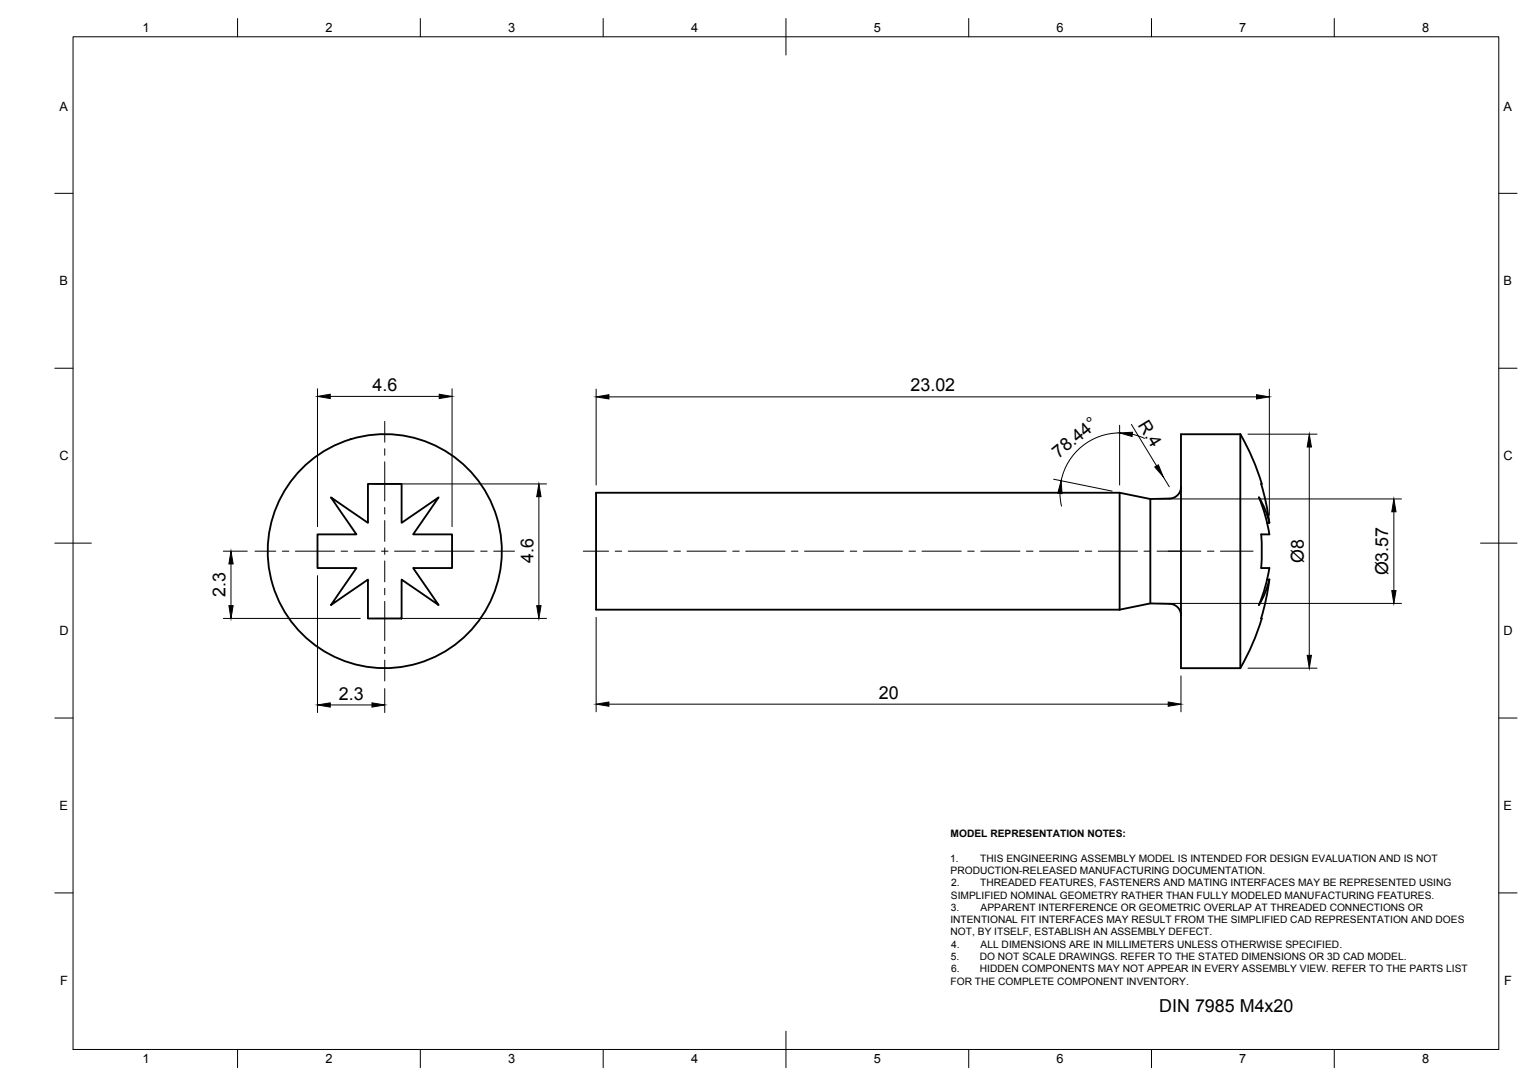
ISO-10303-21;
HEADER;
/* Generated by software containing ST-Developer
 * from STEP Tools, Inc. (www.steptools.com) 
 */

FILE_DESCRIPTION(
/* description */ ('STEP AP214'),
/* implementation_level */ '2;1');

FILE_NAME(
/* name */ 'DIN 7985 M4x20.step',
/* time_stamp */ '2026-10-07T12:18:07-07:00',
/* author */ (''),
/* organization */ (''),
/* preprocessor_version */ 'ST-DEVELOPER v20.2',
/* originating_system */ 'Autodesk Translation Framework v15.15.0.0',
/* authorisation */ '');

FILE_SCHEMA (('AUTOMOTIVE_DESIGN { 1 0 10303 214 3 1 1 }'));
ENDSEC;

DATA;
#10=MECHANICAL_DESIGN_GEOMETRIC_PRESENTATION_REPRESENTATION('',(#123),#62974);
#79=SPHERICAL_SURFACE('',#15475,8.00000000000091);
#99=SHAPE_REPRESENTATION_RELATIONSHIP('SRR','None',#63022,#111);
#111=ADVANCED_BREP_SHAPE_REPRESENTATION('',(#135),#62963);
#123=STYLED_ITEM('',(#63090),#135);
#135=MANIFOLD_SOLID_BREP('Body1',#15193);
#210=FACE_BOUND('',#4662,.T.);
#211=FACE_BOUND('',#4669,.T.);
#342=PLANE('',#15508);
#343=PLANE('',#15509);
#344=PLANE('',#15510);
#345=PLANE('',#15511);
#346=PLANE('',#15512);
#347=PLANE('',#15513);
#348=PLANE('',#15514);
#349=PLANE('',#15515);
#350=PLANE('',#15516);
#351=PLANE('',#15517);
#352=PLANE('',#15518);
#353=PLANE('',#15519);
#354=PLANE('',#15520);
#355=PLANE('',#15521);
#356=PLANE('',#15522);
#357=PLANE('',#15523);
#358=PLANE('',#15524);
#359=PLANE('',#15525);
#360=PLANE('',#15526);
#361=PLANE('',#15527);
#362=PLANE('',#15528);
#363=PLANE('',#15529);
#364=PLANE('',#15530);
#1035=CONICAL_SURFACE('',#15500,1.8001015361136,0.0225322446275356);
#1036=CONICAL_SURFACE('',#15503,1.78525,0.201741568445237);
#1193=LINE('',#33921,#2386);
#1194=LINE('',#33972,#2387);
#1195=LINE('',#33980,#2388);
#1196=LINE('',#33985,#2389);
#1197=LINE('',#33990,#2390);
#1198=LINE('',#33992,#2391);
#1199=LINE('',#33993,#2392);
#1200=LINE('',#33997,#2393);
#1201=LINE('',#33998,#2394);
#1202=LINE('',#33999,#2395);
#1203=LINE('',#34002,#2396);
#1204=LINE('',#34003,#2397);
#1205=LINE('',#34006,#2398);
#1206=LINE('',#34007,#2399);
#1207=LINE('',#34010,#2400);
#1208=LINE('',#34011,#2401);
#1209=LINE('',#34014,#2402);
#1210=LINE('',#34015,#2403);
#1211=LINE('',#34018,#2404);
#1212=LINE('',#34019,#2405);
#1213=LINE('',#34022,#2406);
#1214=LINE('',#34023,#2407);
#1215=LINE('',#34026,#2408);
#1216=LINE('',#34027,#2409);
#1217=LINE('',#34030,#2410);
#1218=LINE('',#34031,#2411);
#1219=LINE('',#34034,#2412);
#1220=LINE('',#34035,#2413);
#1221=LINE('',#34038,#2414);
#1222=LINE('',#34039,#2415);
#1223=LINE('',#34042,#2416);
#1224=LINE('',#34043,#2417);
#1225=LINE('',#34046,#2418);
#1226=LINE('',#34047,#2419);
#1227=LINE('',#34050,#2420);
#1228=LINE('',#34051,#2421);
#1229=LINE('',#34054,#2422);
#1230=LINE('',#34055,#2423);
#1231=LINE('',#34058,#2424);
#1232=LINE('',#34059,#2425);
#1233=LINE('',#34061,#2426);
#1234=LINE('',#34064,#2427);
#1235=LINE('',#34065,#2428);
#1236=LINE('',#34067,#2429);
#2386=VECTOR('',#17366,4.);
#2387=VECTOR('',#17421,1.8001015361136);
#2388=VECTOR('',#17430,1.78525);
#2389=VECTOR('',#17437,2.);
#2390=VECTOR('',#17444,1000.);
#2391=VECTOR('',#17445,1000.);
#2392=VECTOR('',#17446,1000.);
#2393=VECTOR('',#17449,1000.);
#2394=VECTOR('',#17450,1000.);
#2395=VECTOR('',#17451,1000.);
#2396=VECTOR('',#17454,1000.);
#2397=VECTOR('',#17455,1000.);
#2398=VECTOR('',#17458,1000.);
#2399=VECTOR('',#17459,1000.);
#2400=VECTOR('',#17462,1000.);
#2401=VECTOR('',#17463,1000.);
#2402=VECTOR('',#17466,1000.);
#2403=VECTOR('',#17467,1000.);
#2404=VECTOR('',#17470,1000.);
#2405=VECTOR('',#17471,1000.);
#2406=VECTOR('',#17474,1000.);
#2407=VECTOR('',#17475,1000.);
#2408=VECTOR('',#17478,1000.);
#2409=VECTOR('',#17479,1000.);
#2410=VECTOR('',#17482,1000.);
#2411=VECTOR('',#17483,1000.);
#2412=VECTOR('',#17486,1000.);
#2413=VECTOR('',#17487,1000.);
#2414=VECTOR('',#17490,1000.);
#2415=VECTOR('',#17491,1000.);
#2416=VECTOR('',#17494,1000.);
#2417=VECTOR('',#17495,1000.);
#2418=VECTOR('',#17498,1000.);
#2419=VECTOR('',#17499,1000.);
#2420=VECTOR('',#17502,1000.);
#2421=VECTOR('',#17503,1000.);
#2422=VECTOR('',#17506,1000.);
#2423=VECTOR('',#17507,1000.);
#2424=VECTOR('',#17510,1000.);
#2425=VECTOR('',#17511,1000.);
#2426=VECTOR('',#17514,1000.);
#2427=VECTOR('',#17517,1000.);
#2428=VECTOR('',#17518,1000.);
#2429=VECTOR('',#17521,1000.);
#3459=CYLINDRICAL_SURFACE('',#15472,4.);
#3460=CYLINDRICAL_SURFACE('',#15506,2.);
#3777=FACE_OUTER_BOUND('',#4660,.T.);
#3778=FACE_OUTER_BOUND('',#4661,.T.);
#3779=FACE_OUTER_BOUND('',#4663,.T.);
#3780=FACE_OUTER_BOUND('',#4664,.T.);
#3781=FACE_OUTER_BOUND('',#4665,.T.);
#3782=FACE_OUTER_BOUND('',#4666,.T.);
#3783=FACE_OUTER_BOUND('',#4667,.T.);
#3784=FACE_OUTER_BOUND('',#4668,.T.);
#3785=FACE_OUTER_BOUND('',#4670,.T.);
#3786=FACE_OUTER_BOUND('',#4671,.T.);
#3787=FACE_OUTER_BOUND('',#4672,.T.);
#3788=FACE_OUTER_BOUND('',#4673,.T.);
#3789=FACE_OUTER_BOUND('',#4674,.T.);
#3790=FACE_OUTER_BOUND('',#4675,.T.);
#3791=FACE_OUTER_BOUND('',#4676,.T.);
#3792=FACE_OUTER_BOUND('',#4677,.T.);
#3793=FACE_OUTER_BOUND('',#4678,.T.);
#3794=FACE_OUTER_BOUND('',#4679,.T.);
#3795=FACE_OUTER_BOUND('',#4680,.T.);
#3796=FACE_OUTER_BOUND('',#4681,.T.);
#3797=FACE_OUTER_BOUND('',#4682,.T.);
#3798=FACE_OUTER_BOUND('',#4683,.T.);
#3799=FACE_OUTER_BOUND('',#4684,.T.);
#3800=FACE_OUTER_BOUND('',#4685,.T.);
#3801=FACE_OUTER_BOUND('',#4686,.T.);
#3802=FACE_OUTER_BOUND('',#4687,.T.);
#3803=FACE_OUTER_BOUND('',#4688,.T.);
#3804=FACE_OUTER_BOUND('',#4689,.T.);
#3805=FACE_OUTER_BOUND('',#4690,.T.);
#4660=EDGE_LOOP('',(#10207,#10208,#10209,#10210));
#4661=EDGE_LOOP('',(#10211));
#4662=EDGE_LOOP('',(#10212,#10213,#10214,#10215,#10216,#10217,#10218,#10219,
#10220,#10221,#10222,#10223,#10224,#10225,#10226,#10227,#10228,#10229,#10230,
#10231));
#4663=EDGE_LOOP('',(#10232,#10233,#10234,#10235));
#4664=EDGE_LOOP('',(#10236,#10237,#10238,#10239,#10240));
#4665=EDGE_LOOP('',(#10241,#10242,#10243,#10244,#10245,#10246));
#4666=EDGE_LOOP('',(#10247,#10248,#10249,#10250,#10251));
#4667=EDGE_LOOP('',(#10252));
#4668=EDGE_LOOP('',(#10253));
#4669=EDGE_LOOP('',(#10254));
#4670=EDGE_LOOP('',(#10255,#10256,#10257,#10258));
#4671=EDGE_LOOP('',(#10259,#10260,#10261,#10262));
#4672=EDGE_LOOP('',(#10263,#10264,#10265,#10266));
#4673=EDGE_LOOP('',(#10267,#10268,#10269,#10270));
#4674=EDGE_LOOP('',(#10271,#10272,#10273,#10274));
#4675=EDGE_LOOP('',(#10275,#10276,#10277,#10278));
#4676=EDGE_LOOP('',(#10279,#10280,#10281,#10282));
#4677=EDGE_LOOP('',(#10283,#10284,#10285,#10286));
#4678=EDGE_LOOP('',(#10287,#10288,#10289,#10290));
#4679=EDGE_LOOP('',(#10291,#10292,#10293,#10294));
#4680=EDGE_LOOP('',(#10295,#10296,#10297,#10298));
#4681=EDGE_LOOP('',(#10299,#10300,#10301,#10302));
#4682=EDGE_LOOP('',(#10303,#10304,#10305,#10306));
#4683=EDGE_LOOP('',(#10307,#10308,#10309,#10310));
#4684=EDGE_LOOP('',(#10311,#10312,#10313,#10314));
#4685=EDGE_LOOP('',(#10315,#10316,#10317,#10318));
#4686=EDGE_LOOP('',(#10319,#10320,#10321,#10322));
#4687=EDGE_LOOP('',(#10323,#10324,#10325,#10326));
#4688=EDGE_LOOP('',(#10327,#10328,#10329,#10330,#10331,#10332,#10333,#10334,
#10335,#10336,#10337,#10338,#10339,#10340,#10341,#10342,#10343,#10344,#10345,
#10346));
#4689=EDGE_LOOP('',(#10347,#10348,#10349,#10350));
#4690=EDGE_LOOP('',(#10351,#10352,#10353,#10354));
#5553=CIRCLE('',#15473,4.);
#5554=CIRCLE('',#15474,4.);
#5555=CIRCLE('',#15476,7.66224510179708);
#5556=CIRCLE('',#15477,7.97930918062551);
#5557=CIRCLE('',#15478,7.98595584236444);
#5558=CIRCLE('',#15479,7.98595584236446);
#5559=CIRCLE('',#15480,7.97930918062549);
#5560=CIRCLE('',#15481,7.66224510179716);
#5561=CIRCLE('',#15482,7.97930918062553);
#5562=CIRCLE('',#15483,7.98595584236444);
#5563=CIRCLE('',#15484,7.98595584236446);
#5564=CIRCLE('',#15485,7.97930918062551);
#5565=CIRCLE('',#15486,7.66224510179724);
#5566=CIRCLE('',#15487,7.97930918062551);
#5567=CIRCLE('',#15488,7.98595584236446);
#5568=CIRCLE('',#15489,7.98595584236444);
#5569=CIRCLE('',#15490,7.97930918062553);
#5570=CIRCLE('',#15491,7.66224510179716);
#5571=CIRCLE('',#15492,7.97930918062549);
#5572=CIRCLE('',#15493,7.98595584236446);
#5573=CIRCLE('',#15494,7.98595584236444);
#5574=CIRCLE('',#15495,7.97930918062551);
#5575=CIRCLE('',#15497,2.2);
#5576=CIRCLE('',#15498,0.40000000000004);
#5577=CIRCLE('',#15499,1.8001015361136);
#5578=CIRCLE('',#15501,1.78525);
#5579=CIRCLE('',#15502,1.78525);
#5580=CIRCLE('',#15504,2.);
#5581=CIRCLE('',#15505,2.);
#5582=CIRCLE('',#15507,2.);
#6337=VERTEX_POINT('',#33918);
#6338=VERTEX_POINT('',#33920);
#6339=VERTEX_POINT('',#33924);
#6340=VERTEX_POINT('',#33925);
#6341=VERTEX_POINT('',#33927);
#6342=VERTEX_POINT('',#33929);
#6343=VERTEX_POINT('',#33931);
#6344=VERTEX_POINT('',#33933);
#6345=VERTEX_POINT('',#33935);
#6346=VERTEX_POINT('',#33937);
#6347=VERTEX_POINT('',#33939);
#6348=VERTEX_POINT('',#33941);
#6349=VERTEX_POINT('',#33943);
#6350=VERTEX_POINT('',#33945);
#6351=VERTEX_POINT('',#33947);
#6352=VERTEX_POINT('',#33949);
#6353=VERTEX_POINT('',#33951);
#6354=VERTEX_POINT('',#33953);
#6355=VERTEX_POINT('',#33955);
#6356=VERTEX_POINT('',#33957);
#6357=VERTEX_POINT('',#33959);
#6358=VERTEX_POINT('',#33961);
#6359=VERTEX_POINT('',#33965);
#6360=VERTEX_POINT('',#33967);
#6361=VERTEX_POINT('',#33971);
#6362=VERTEX_POINT('',#33973);
#6363=VERTEX_POINT('',#33977);
#6364=VERTEX_POINT('',#33978);
#6365=VERTEX_POINT('',#33983);
#6366=VERTEX_POINT('',#33989);
#6367=VERTEX_POINT('',#33991);
#6368=VERTEX_POINT('',#33995);
#6369=VERTEX_POINT('',#33996);
#6370=VERTEX_POINT('',#34001);
#6371=VERTEX_POINT('',#34005);
#6372=VERTEX_POINT('',#34009);
#6373=VERTEX_POINT('',#34013);
#6374=VERTEX_POINT('',#34017);
#6375=VERTEX_POINT('',#34021);
#6376=VERTEX_POINT('',#34025);
#6377=VERTEX_POINT('',#34029);
#6378=VERTEX_POINT('',#34033);
#6379=VERTEX_POINT('',#34037);
#6380=VERTEX_POINT('',#34041);
#6381=VERTEX_POINT('',#34045);
#6382=VERTEX_POINT('',#34049);
#6383=VERTEX_POINT('',#34053);
#6384=VERTEX_POINT('',#34057);
#6385=VERTEX_POINT('',#34063);
#7810=EDGE_CURVE('',#6337,#6337,#5553,.T.);
#7811=EDGE_CURVE('',#6337,#6338,#1193,.T.);
#7812=EDGE_CURVE('',#6338,#6338,#5554,.T.);
#7813=EDGE_CURVE('',#6339,#6340,#5555,.T.);
#7814=EDGE_CURVE('',#6340,#6341,#5556,.T.);
#7815=EDGE_CURVE('',#6341,#6342,#5557,.T.);
#7816=EDGE_CURVE('',#6342,#6343,#5558,.T.);
#7817=EDGE_CURVE('',#6343,#6344,#5559,.T.);
#7818=EDGE_CURVE('',#6344,#6345,#5560,.T.);
#7819=EDGE_CURVE('',#6345,#6346,#5561,.T.);
#7820=EDGE_CURVE('',#6346,#6347,#5562,.T.);
#7821=EDGE_CURVE('',#6347,#6348,#5563,.T.);
#7822=EDGE_CURVE('',#6348,#6349,#5564,.T.);
#7823=EDGE_CURVE('',#6349,#6350,#5565,.T.);
#7824=EDGE_CURVE('',#6350,#6351,#5566,.T.);
#7825=EDGE_CURVE('',#6351,#6352,#5567,.T.);
#7826=EDGE_CURVE('',#6352,#6353,#5568,.T.);
#7827=EDGE_CURVE('',#6353,#6354,#5569,.T.);
#7828=EDGE_CURVE('',#6354,#6355,#5570,.T.);
#7829=EDGE_CURVE('',#6355,#6356,#5571,.T.);
#7830=EDGE_CURVE('',#6356,#6357,#5572,.T.);
#7831=EDGE_CURVE('',#6357,#6358,#5573,.T.);
#7832=EDGE_CURVE('',#6358,#6339,#5574,.T.);
#7833=EDGE_CURVE('',#6359,#6359,#5575,.T.);
#7834=EDGE_CURVE('',#6359,#6360,#5576,.T.);
#7835=EDGE_CURVE('',#6360,#6360,#5577,.T.);
#7836=EDGE_CURVE('',#6360,#6361,#1194,.T.);
#7837=EDGE_CURVE('',#6361,#6362,#5578,.T.);
#7838=EDGE_CURVE('',#6362,#6361,#5579,.T.);
#7839=EDGE_CURVE('',#6363,#6364,#5580,.T.);
#7840=EDGE_CURVE('',#6364,#6362,#1195,.T.);
#7841=EDGE_CURVE('',#6364,#6363,#5581,.T.);
#7842=EDGE_CURVE('',#6365,#6365,#5582,.T.);
#7843=EDGE_CURVE('',#6365,#6363,#1196,.T.);
#7844=EDGE_CURVE('',#6343,#6366,#1197,.T.);
#7845=EDGE_CURVE('',#6366,#6367,#1198,.T.);
#7846=EDGE_CURVE('',#6344,#6367,#1199,.T.);
#7847=EDGE_CURVE('',#6368,#6369,#1200,.T.);
#7848=EDGE_CURVE('',#6369,#6341,#1201,.T.);
#7849=EDGE_CURVE('',#6340,#6368,#1202,.T.);
#7850=EDGE_CURVE('',#6339,#6370,#1203,.T.);
#7851=EDGE_CURVE('',#6370,#6368,#1204,.T.);
#7852=EDGE_CURVE('',#6358,#6371,#1205,.T.);
#7853=EDGE_CURVE('',#6371,#6370,#1206,.T.);
#7854=EDGE_CURVE('',#6357,#6372,#1207,.T.);
#7855=EDGE_CURVE('',#6372,#6371,#1208,.T.);
#7856=EDGE_CURVE('',#6373,#6356,#1209,.T.);
#7857=EDGE_CURVE('',#6373,#6372,#1210,.T.);
#7858=EDGE_CURVE('',#6374,#6373,#1211,.T.);
#7859=EDGE_CURVE('',#6355,#6374,#1212,.T.);
#7860=EDGE_CURVE('',#6354,#6375,#1213,.T.);
#7861=EDGE_CURVE('',#6375,#6374,#1214,.T.);
#7862=EDGE_CURVE('',#6353,#6376,#1215,.T.);
#7863=EDGE_CURVE('',#6376,#6375,#1216,.T.);
#7864=EDGE_CURVE('',#6352,#6377,#1217,.T.);
#7865=EDGE_CURVE('',#6377,#6376,#1218,.T.);
#7866=EDGE_CURVE('',#6378,#6351,#1219,.T.);
#7867=EDGE_CURVE('',#6378,#6377,#1220,.T.);
#7868=EDGE_CURVE('',#6379,#6378,#1221,.T.);
#7869=EDGE_CURVE('',#6350,#6379,#1222,.T.);
#7870=EDGE_CURVE('',#6349,#6380,#1223,.T.);
#7871=EDGE_CURVE('',#6380,#6379,#1224,.T.);
#7872=EDGE_CURVE('',#6348,#6381,#1225,.T.);
#7873=EDGE_CURVE('',#6381,#6380,#1226,.T.);
#7874=EDGE_CURVE('',#6347,#6382,#1227,.T.);
#7875=EDGE_CURVE('',#6382,#6381,#1228,.T.);
#7876=EDGE_CURVE('',#6383,#6346,#1229,.T.);
#7877=EDGE_CURVE('',#6383,#6382,#1230,.T.);
#7878=EDGE_CURVE('',#6384,#6383,#1231,.T.);
#7879=EDGE_CURVE('',#6345,#6384,#1232,.T.);
#7880=EDGE_CURVE('',#6367,#6384,#1233,.T.);
#7881=EDGE_CURVE('',#6369,#6385,#1234,.T.);
#7882=EDGE_CURVE('',#6385,#6366,#1235,.T.);
#7883=EDGE_CURVE('',#6342,#6385,#1236,.T.);
#10207=ORIENTED_EDGE('',*,*,#7810,.T.);
#10208=ORIENTED_EDGE('',*,*,#7811,.T.);
#10209=ORIENTED_EDGE('',*,*,#7812,.F.);
#10210=ORIENTED_EDGE('',*,*,#7811,.F.);
#10211=ORIENTED_EDGE('',*,*,#7812,.T.);
#10212=ORIENTED_EDGE('',*,*,#7813,.T.);
#10213=ORIENTED_EDGE('',*,*,#7814,.T.);
#10214=ORIENTED_EDGE('',*,*,#7815,.T.);
#10215=ORIENTED_EDGE('',*,*,#7816,.T.);
#10216=ORIENTED_EDGE('',*,*,#7817,.T.);
#10217=ORIENTED_EDGE('',*,*,#7818,.T.);
#10218=ORIENTED_EDGE('',*,*,#7819,.T.);
#10219=ORIENTED_EDGE('',*,*,#7820,.T.);
#10220=ORIENTED_EDGE('',*,*,#7821,.T.);
#10221=ORIENTED_EDGE('',*,*,#7822,.T.);
#10222=ORIENTED_EDGE('',*,*,#7823,.T.);
#10223=ORIENTED_EDGE('',*,*,#7824,.T.);
#10224=ORIENTED_EDGE('',*,*,#7825,.T.);
#10225=ORIENTED_EDGE('',*,*,#7826,.T.);
#10226=ORIENTED_EDGE('',*,*,#7827,.T.);
#10227=ORIENTED_EDGE('',*,*,#7828,.T.);
#10228=ORIENTED_EDGE('',*,*,#7829,.T.);
#10229=ORIENTED_EDGE('',*,*,#7830,.T.);
#10230=ORIENTED_EDGE('',*,*,#7831,.T.);
#10231=ORIENTED_EDGE('',*,*,#7832,.T.);
#10232=ORIENTED_EDGE('',*,*,#7833,.T.);
#10233=ORIENTED_EDGE('',*,*,#7834,.T.);
#10234=ORIENTED_EDGE('',*,*,#7835,.T.);
#10235=ORIENTED_EDGE('',*,*,#7834,.F.);
#10236=ORIENTED_EDGE('',*,*,#7835,.F.);
#10237=ORIENTED_EDGE('',*,*,#7836,.T.);
#10238=ORIENTED_EDGE('',*,*,#7837,.T.);
#10239=ORIENTED_EDGE('',*,*,#7838,.T.);
#10240=ORIENTED_EDGE('',*,*,#7836,.F.);
#10241=ORIENTED_EDGE('',*,*,#7839,.T.);
#10242=ORIENTED_EDGE('',*,*,#7840,.T.);
#10243=ORIENTED_EDGE('',*,*,#7837,.F.);
#10244=ORIENTED_EDGE('',*,*,#7838,.F.);
#10245=ORIENTED_EDGE('',*,*,#7840,.F.);
#10246=ORIENTED_EDGE('',*,*,#7841,.T.);
#10247=ORIENTED_EDGE('',*,*,#7842,.T.);
#10248=ORIENTED_EDGE('',*,*,#7843,.T.);
#10249=ORIENTED_EDGE('',*,*,#7841,.F.);
#10250=ORIENTED_EDGE('',*,*,#7839,.F.);
#10251=ORIENTED_EDGE('',*,*,#7843,.F.);
#10252=ORIENTED_EDGE('',*,*,#7842,.F.);
#10253=ORIENTED_EDGE('',*,*,#7810,.F.);
#10254=ORIENTED_EDGE('',*,*,#7833,.F.);
#10255=ORIENTED_EDGE('',*,*,#7817,.F.);
#10256=ORIENTED_EDGE('',*,*,#7844,.T.);
#10257=ORIENTED_EDGE('',*,*,#7845,.T.);
#10258=ORIENTED_EDGE('',*,*,#7846,.F.);
#10259=ORIENTED_EDGE('',*,*,#7847,.T.);
#10260=ORIENTED_EDGE('',*,*,#7848,.T.);
#10261=ORIENTED_EDGE('',*,*,#7814,.F.);
#10262=ORIENTED_EDGE('',*,*,#7849,.T.);
#10263=ORIENTED_EDGE('',*,*,#7850,.T.);
#10264=ORIENTED_EDGE('',*,*,#7851,.T.);
#10265=ORIENTED_EDGE('',*,*,#7849,.F.);
#10266=ORIENTED_EDGE('',*,*,#7813,.F.);
#10267=ORIENTED_EDGE('',*,*,#7832,.F.);
#10268=ORIENTED_EDGE('',*,*,#7852,.T.);
#10269=ORIENTED_EDGE('',*,*,#7853,.T.);
#10270=ORIENTED_EDGE('',*,*,#7850,.F.);
#10271=ORIENTED_EDGE('',*,*,#7854,.T.);
#10272=ORIENTED_EDGE('',*,*,#7855,.T.);
#10273=ORIENTED_EDGE('',*,*,#7852,.F.);
#10274=ORIENTED_EDGE('',*,*,#7831,.F.);
#10275=ORIENTED_EDGE('',*,*,#7856,.F.);
#10276=ORIENTED_EDGE('',*,*,#7857,.T.);
#10277=ORIENTED_EDGE('',*,*,#7854,.F.);
#10278=ORIENTED_EDGE('',*,*,#7830,.F.);
#10279=ORIENTED_EDGE('',*,*,#7858,.T.);
#10280=ORIENTED_EDGE('',*,*,#7856,.T.);
#10281=ORIENTED_EDGE('',*,*,#7829,.F.);
#10282=ORIENTED_EDGE('',*,*,#7859,.T.);
#10283=ORIENTED_EDGE('',*,*,#7860,.T.);
#10284=ORIENTED_EDGE('',*,*,#7861,.T.);
#10285=ORIENTED_EDGE('',*,*,#7859,.F.);
#10286=ORIENTED_EDGE('',*,*,#7828,.F.);
#10287=ORIENTED_EDGE('',*,*,#7827,.F.);
#10288=ORIENTED_EDGE('',*,*,#7862,.T.);
#10289=ORIENTED_EDGE('',*,*,#7863,.T.);
#10290=ORIENTED_EDGE('',*,*,#7860,.F.);
#10291=ORIENTED_EDGE('',*,*,#7864,.T.);
#10292=ORIENTED_EDGE('',*,*,#7865,.T.);
#10293=ORIENTED_EDGE('',*,*,#7862,.F.);
#10294=ORIENTED_EDGE('',*,*,#7826,.F.);
#10295=ORIENTED_EDGE('',*,*,#7866,.F.);
#10296=ORIENTED_EDGE('',*,*,#7867,.T.);
#10297=ORIENTED_EDGE('',*,*,#7864,.F.);
#10298=ORIENTED_EDGE('',*,*,#7825,.F.);
#10299=ORIENTED_EDGE('',*,*,#7868,.T.);
#10300=ORIENTED_EDGE('',*,*,#7866,.T.);
#10301=ORIENTED_EDGE('',*,*,#7824,.F.);
#10302=ORIENTED_EDGE('',*,*,#7869,.T.);
#10303=ORIENTED_EDGE('',*,*,#7870,.T.);
#10304=ORIENTED_EDGE('',*,*,#7871,.T.);
#10305=ORIENTED_EDGE('',*,*,#7869,.F.);
#10306=ORIENTED_EDGE('',*,*,#7823,.F.);
#10307=ORIENTED_EDGE('',*,*,#7822,.F.);
#10308=ORIENTED_EDGE('',*,*,#7872,.T.);
#10309=ORIENTED_EDGE('',*,*,#7873,.T.);
#10310=ORIENTED_EDGE('',*,*,#7870,.F.);
#10311=ORIENTED_EDGE('',*,*,#7874,.T.);
#10312=ORIENTED_EDGE('',*,*,#7875,.T.);
#10313=ORIENTED_EDGE('',*,*,#7872,.F.);
#10314=ORIENTED_EDGE('',*,*,#7821,.F.);
#10315=ORIENTED_EDGE('',*,*,#7876,.F.);
#10316=ORIENTED_EDGE('',*,*,#7877,.T.);
#10317=ORIENTED_EDGE('',*,*,#7874,.F.);
#10318=ORIENTED_EDGE('',*,*,#7820,.F.);
#10319=ORIENTED_EDGE('',*,*,#7878,.T.);
#10320=ORIENTED_EDGE('',*,*,#7876,.T.);
#10321=ORIENTED_EDGE('',*,*,#7819,.F.);
#10322=ORIENTED_EDGE('',*,*,#7879,.T.);
#10323=ORIENTED_EDGE('',*,*,#7846,.T.);
#10324=ORIENTED_EDGE('',*,*,#7880,.T.);
#10325=ORIENTED_EDGE('',*,*,#7879,.F.);
#10326=ORIENTED_EDGE('',*,*,#7818,.F.);
#10327=ORIENTED_EDGE('',*,*,#7881,.F.);
#10328=ORIENTED_EDGE('',*,*,#7847,.F.);
#10329=ORIENTED_EDGE('',*,*,#7851,.F.);
#10330=ORIENTED_EDGE('',*,*,#7853,.F.);
#10331=ORIENTED_EDGE('',*,*,#7855,.F.);
#10332=ORIENTED_EDGE('',*,*,#7857,.F.);
#10333=ORIENTED_EDGE('',*,*,#7858,.F.);
#10334=ORIENTED_EDGE('',*,*,#7861,.F.);
#10335=ORIENTED_EDGE('',*,*,#7863,.F.);
#10336=ORIENTED_EDGE('',*,*,#7865,.F.);
#10337=ORIENTED_EDGE('',*,*,#7867,.F.);
#10338=ORIENTED_EDGE('',*,*,#7868,.F.);
#10339=ORIENTED_EDGE('',*,*,#7871,.F.);
#10340=ORIENTED_EDGE('',*,*,#7873,.F.);
#10341=ORIENTED_EDGE('',*,*,#7875,.F.);
#10342=ORIENTED_EDGE('',*,*,#7877,.F.);
#10343=ORIENTED_EDGE('',*,*,#7878,.F.);
#10344=ORIENTED_EDGE('',*,*,#7880,.F.);
#10345=ORIENTED_EDGE('',*,*,#7845,.F.);
#10346=ORIENTED_EDGE('',*,*,#7882,.F.);
#10347=ORIENTED_EDGE('',*,*,#7883,.T.);
#10348=ORIENTED_EDGE('',*,*,#7882,.T.);
#10349=ORIENTED_EDGE('',*,*,#7844,.F.);
#10350=ORIENTED_EDGE('',*,*,#7816,.F.);
#10351=ORIENTED_EDGE('',*,*,#7848,.F.);
#10352=ORIENTED_EDGE('',*,*,#7881,.T.);
#10353=ORIENTED_EDGE('',*,*,#7883,.F.);
#10354=ORIENTED_EDGE('',*,*,#7815,.F.);
#14255=TOROIDAL_SURFACE('',#15496,2.2,0.40000000000004);
#14412=ADVANCED_FACE('',(#3777),#3459,.T.);
#14413=ADVANCED_FACE('',(#3778,#210),#79,.T.);
#14414=ADVANCED_FACE('',(#3779),#14255,.F.);
#14415=ADVANCED_FACE('',(#3780),#1035,.T.);
#14416=ADVANCED_FACE('',(#3781),#1036,.T.);
#14417=ADVANCED_FACE('',(#3782),#3460,.T.);
#14418=ADVANCED_FACE('',(#3783),#342,.T.);
#14419=ADVANCED_FACE('',(#3784,#211),#343,.T.);
#14420=ADVANCED_FACE('',(#3785),#344,.F.);
#14421=ADVANCED_FACE('',(#3786),#345,.F.);
#14422=ADVANCED_FACE('',(#3787),#346,.F.);
#14423=ADVANCED_FACE('',(#3788),#347,.F.);
#14424=ADVANCED_FACE('',(#3789),#348,.F.);
#14425=ADVANCED_FACE('',(#3790),#349,.F.);
#14426=ADVANCED_FACE('',(#3791),#350,.F.);
#14427=ADVANCED_FACE('',(#3792),#351,.F.);
#14428=ADVANCED_FACE('',(#3793),#352,.F.);
#14429=ADVANCED_FACE('',(#3794),#353,.F.);
#14430=ADVANCED_FACE('',(#3795),#354,.F.);
#14431=ADVANCED_FACE('',(#3796),#355,.F.);
#14432=ADVANCED_FACE('',(#3797),#356,.F.);
#14433=ADVANCED_FACE('',(#3798),#357,.F.);
#14434=ADVANCED_FACE('',(#3799),#358,.F.);
#14435=ADVANCED_FACE('',(#3800),#359,.F.);
#14436=ADVANCED_FACE('',(#3801),#360,.F.);
#14437=ADVANCED_FACE('',(#3802),#361,.F.);
#14438=ADVANCED_FACE('',(#3803),#362,.F.);
#14439=ADVANCED_FACE('',(#3804),#363,.F.);
#14440=ADVANCED_FACE('',(#3805),#364,.F.);
#15193=CLOSED_SHELL('',(#14412,#14413,#14414,#14415,#14416,#14417,#14418,
#14419,#14420,#14421,#14422,#14423,#14424,#14425,#14426,#14427,#14428,#14429,
#14430,#14431,#14432,#14433,#14434,#14435,#14436,#14437,#14438,#14439,#14440));
#15471=AXIS2_PLACEMENT_3D('',#33916,#17360,#17361);
#15472=AXIS2_PLACEMENT_3D('',#33917,#17362,#17363);
#15473=AXIS2_PLACEMENT_3D('',#33919,#17364,#17365);
#15474=AXIS2_PLACEMENT_3D('',#33922,#17367,#17368);
#15475=AXIS2_PLACEMENT_3D('',#33923,#17369,#17370);
#15476=AXIS2_PLACEMENT_3D('',#33926,#17371,#17372);
#15477=AXIS2_PLACEMENT_3D('',#33928,#17373,#17374);
#15478=AXIS2_PLACEMENT_3D('',#33930,#17375,#17376);
#15479=AXIS2_PLACEMENT_3D('',#33932,#17377,#17378);
#15480=AXIS2_PLACEMENT_3D('',#33934,#17379,#17380);
#15481=AXIS2_PLACEMENT_3D('',#33936,#17381,#17382);
#15482=AXIS2_PLACEMENT_3D('',#33938,#17383,#17384);
#15483=AXIS2_PLACEMENT_3D('',#33940,#17385,#17386);
#15484=AXIS2_PLACEMENT_3D('',#33942,#17387,#17388);
#15485=AXIS2_PLACEMENT_3D('',#33944,#17389,#17390);
#15486=AXIS2_PLACEMENT_3D('',#33946,#17391,#17392);
#15487=AXIS2_PLACEMENT_3D('',#33948,#17393,#17394);
#15488=AXIS2_PLACEMENT_3D('',#33950,#17395,#17396);
#15489=AXIS2_PLACEMENT_3D('',#33952,#17397,#17398);
#15490=AXIS2_PLACEMENT_3D('',#33954,#17399,#17400);
#15491=AXIS2_PLACEMENT_3D('',#33956,#17401,#17402);
#15492=AXIS2_PLACEMENT_3D('',#33958,#17403,#17404);
#15493=AXIS2_PLACEMENT_3D('',#33960,#17405,#17406);
#15494=AXIS2_PLACEMENT_3D('',#33962,#17407,#17408);
#15495=AXIS2_PLACEMENT_3D('',#33963,#17409,#17410);
#15496=AXIS2_PLACEMENT_3D('',#33964,#17411,#17412);
#15497=AXIS2_PLACEMENT_3D('',#33966,#17413,#17414);
#15498=AXIS2_PLACEMENT_3D('',#33968,#17415,#17416);
#15499=AXIS2_PLACEMENT_3D('',#33969,#17417,#17418);
#15500=AXIS2_PLACEMENT_3D('',#33970,#17419,#17420);
#15501=AXIS2_PLACEMENT_3D('',#33974,#17422,#17423);
#15502=AXIS2_PLACEMENT_3D('',#33975,#17424,#17425);
#15503=AXIS2_PLACEMENT_3D('',#33976,#17426,#17427);
#15504=AXIS2_PLACEMENT_3D('',#33979,#17428,#17429);
#15505=AXIS2_PLACEMENT_3D('',#33981,#17431,#17432);
#15506=AXIS2_PLACEMENT_3D('',#33982,#17433,#17434);
#15507=AXIS2_PLACEMENT_3D('',#33984,#17435,#17436);
#15508=AXIS2_PLACEMENT_3D('',#33986,#17438,#17439);
#15509=AXIS2_PLACEMENT_3D('',#33987,#17440,#17441);
#15510=AXIS2_PLACEMENT_3D('',#33988,#17442,#17443);
#15511=AXIS2_PLACEMENT_3D('',#33994,#17447,#17448);
#15512=AXIS2_PLACEMENT_3D('',#34000,#17452,#17453);
#15513=AXIS2_PLACEMENT_3D('',#34004,#17456,#17457);
#15514=AXIS2_PLACEMENT_3D('',#34008,#17460,#17461);
#15515=AXIS2_PLACEMENT_3D('',#34012,#17464,#17465);
#15516=AXIS2_PLACEMENT_3D('',#34016,#17468,#17469);
#15517=AXIS2_PLACEMENT_3D('',#34020,#17472,#17473);
#15518=AXIS2_PLACEMENT_3D('',#34024,#17476,#17477);
#15519=AXIS2_PLACEMENT_3D('',#34028,#17480,#17481);
#15520=AXIS2_PLACEMENT_3D('',#34032,#17484,#17485);
#15521=AXIS2_PLACEMENT_3D('',#34036,#17488,#17489);
#15522=AXIS2_PLACEMENT_3D('',#34040,#17492,#17493);
#15523=AXIS2_PLACEMENT_3D('',#34044,#17496,#17497);
#15524=AXIS2_PLACEMENT_3D('',#34048,#17500,#17501);
#15525=AXIS2_PLACEMENT_3D('',#34052,#17504,#17505);
#15526=AXIS2_PLACEMENT_3D('',#34056,#17508,#17509);
#15527=AXIS2_PLACEMENT_3D('',#34060,#17512,#17513);
#15528=AXIS2_PLACEMENT_3D('',#34062,#17515,#17516);
#15529=AXIS2_PLACEMENT_3D('',#34066,#17519,#17520);
#15530=AXIS2_PLACEMENT_3D('',#34068,#17522,#17523);
#17360=DIRECTION('axis',(0.,0.,1.));
#17361=DIRECTION('refdir',(1.,0.,0.));
#17362=DIRECTION('center_axis',(0.4309815049242,0.768119965562789,-0.473546894105633));
#17363=DIRECTION('ref_axis',(0.473546894105632,0.254189745109286,0.843291712614434));
#17364=DIRECTION('center_axis',(-0.4309815049242,-0.768119965562789,0.473546894105633));
#17365=DIRECTION('ref_axis',(0.473546894105632,0.254189745109287,0.843291712614434));
#17366=DIRECTION('',(-0.4309815049242,-0.768119965562789,0.473546894105633));
#17367=DIRECTION('center_axis',(-0.4309815049242,-0.768119965562789,0.473546894105633));
#17368=DIRECTION('ref_axis',(0.473546894105632,0.254189745109287,0.843291712614434));
#17369=DIRECTION('center_axis',(-0.473546894105632,-0.254189745109287,-0.843291712614434));
#17370=DIRECTION('ref_axis',(-0.768119965562789,0.587689792309766,0.254189745109285));
#17371=DIRECTION('center_axis',(-0.76811996556279,0.587689792309766,0.254189745109285));
#17372=DIRECTION('ref_axis',(0.473546894105632,0.254189745109286,0.843291712614434));
#17373=DIRECTION('center_axis',(0.473546894105632,0.254189745109287,0.843291712614434));
#17374=DIRECTION('ref_axis',(0.4309815049242,0.768119965562789,-0.473546894105633));
#17375=DIRECTION('center_axis',(-0.901241018937803,0.340275210200539,-0.268286054626271));
#17376=DIRECTION('ref_axis',(-0.044939606108901,0.542406212931598,0.838913542610905));
#17377=DIRECTION('center_axis',(0.825384593743779,-0.123480199588392,0.550901908437453));
#17378=DIRECTION('ref_axis',(0.364685089938824,-0.628286844373994,-0.687212067969474));
#17379=DIRECTION('center_axis',(-0.76811996556279,0.587689792309766,0.254189745109285));
#17380=DIRECTION('ref_axis',(0.473546894105632,0.254189745109287,0.843291712614434));
#17381=DIRECTION('center_axis',(0.473546894105632,0.254189745109287,0.843291712614434));
#17382=DIRECTION('ref_axis',(0.4309815049242,0.768119965562789,-0.473546894105633));
#17383=DIRECTION('center_axis',(0.76811996556279,-0.587689792309766,-0.254189745109285));
#17384=DIRECTION('ref_axis',(-0.473546894105632,-0.254189745109286,-0.843291712614434));
#17385=DIRECTION('center_axis',(-0.0449396061089009,0.542406212931599,0.838913542610905));
#17386=DIRECTION('ref_axis',(0.901241018937803,-0.340275210200539,0.268286054626271));
#17387=DIRECTION('center_axis',(0.364685089938824,-0.628286844373994,-0.687212067969474));
#17388=DIRECTION('ref_axis',(-0.825384593743779,0.123480199588392,-0.550901908437453));
#17389=DIRECTION('center_axis',(0.473546894105632,0.254189745109287,0.843291712614434));
#17390=DIRECTION('ref_axis',(0.4309815049242,0.768119965562789,-0.473546894105633));
#17391=DIRECTION('center_axis',(0.76811996556279,-0.587689792309766,-0.254189745109285));
#17392=DIRECTION('ref_axis',(-0.473546894105632,-0.254189745109287,-0.843291712614434));
#17393=DIRECTION('center_axis',(-0.473546894105632,-0.254189745109287,-0.843291712614434));
#17394=DIRECTION('ref_axis',(-0.4309815049242,-0.768119965562789,0.473546894105633));
#17395=DIRECTION('center_axis',(0.901241018937803,-0.340275210200539,0.268286054626271));
#17396=DIRECTION('ref_axis',(0.0449396061089008,-0.542406212931599,-0.838913542610904));
#17397=DIRECTION('center_axis',(-0.825384593743779,0.123480199588392,-0.550901908437453));
#17398=DIRECTION('ref_axis',(-0.364685089938825,0.628286844373993,0.687212067969474));
#17399=DIRECTION('center_axis',(0.76811996556279,-0.587689792309766,-0.254189745109285));
#17400=DIRECTION('ref_axis',(-0.473546894105632,-0.254189745109286,-0.843291712614434));
#17401=DIRECTION('center_axis',(-0.473546894105632,-0.254189745109287,-0.843291712614434));
#17402=DIRECTION('ref_axis',(-0.4309815049242,-0.768119965562789,0.473546894105633));
#17403=DIRECTION('center_axis',(-0.76811996556279,0.587689792309766,0.254189745109285));
#17404=DIRECTION('ref_axis',(0.473546894105632,0.254189745109287,0.843291712614434));
#17405=DIRECTION('center_axis',(0.0449396061089009,-0.542406212931599,-0.838913542610905));
#17406=DIRECTION('ref_axis',(-0.901241018937802,0.34027521020054,-0.268286054626271));
#17407=DIRECTION('center_axis',(-0.364685089938824,0.628286844373994,0.687212067969474));
#17408=DIRECTION('ref_axis',(0.825384593743779,-0.123480199588392,0.550901908437452));
#17409=DIRECTION('center_axis',(-0.473546894105632,-0.254189745109287,-0.843291712614434));
#17410=DIRECTION('ref_axis',(-0.4309815049242,-0.768119965562789,0.473546894105633));
#17411=DIRECTION('center_axis',(-0.4309815049242,-0.768119965562789,0.473546894105633));
#17412=DIRECTION('ref_axis',(0.473546894105633,0.254189745109285,0.843291712614434));
#17413=DIRECTION('center_axis',(0.4309815049242,0.768119965562789,-0.473546894105633));
#17414=DIRECTION('ref_axis',(0.473546894105631,0.254189745109287,0.843291712614434));
#17415=DIRECTION('center_axis',(-0.768119965562789,0.587689792309766,0.254189745109285));
#17416=DIRECTION('ref_axis',(-0.473546894105632,-0.254189745109286,-0.843291712614434));
#17417=DIRECTION('center_axis',(-0.4309815049242,-0.768119965562789,0.473546894105633));
#17418=DIRECTION('ref_axis',(0.473546894105632,0.254189745109287,0.843291712614434));
#17419=DIRECTION('center_axis',(-0.4309815049242,-0.768119965562789,0.473546894105633));
#17420=DIRECTION('ref_axis',(0.473546894105632,0.254189745109287,0.843291712614434));
#17421=DIRECTION('',(0.441541276070288,0.773651966662426,-0.454427041455041));
#17422=DIRECTION('center_axis',(-0.4309815049242,-0.768119965562789,0.473546894105633));
#17423=DIRECTION('ref_axis',(0.473546894105631,0.254189745109287,0.843291712614434));
#17424=DIRECTION('center_axis',(-0.4309815049242,-0.768119965562789,0.473546894105633));
#17425=DIRECTION('ref_axis',(0.473546894105631,0.254189745109287,0.843291712614434));
#17426=DIRECTION('center_axis',(0.4309815049242,0.768119965562789,-0.473546894105633));
#17427=DIRECTION('ref_axis',(-0.473546894105631,-0.254189745109287,-0.843291712614434));
#17428=DIRECTION('center_axis',(-0.4309815049242,-0.768119965562789,0.473546894105633));
#17429=DIRECTION('ref_axis',(0.473546894105632,0.254189745109286,0.843291712614434));
#17430=DIRECTION('',(-0.517128186590923,-0.803475292167847,0.29496761433923));
#17431=DIRECTION('center_axis',(-0.4309815049242,-0.768119965562789,0.473546894105633));
#17432=DIRECTION('ref_axis',(0.473546894105632,0.254189745109286,0.843291712614434));
#17433=DIRECTION('center_axis',(0.4309815049242,0.768119965562789,-0.473546894105633));
#17434=DIRECTION('ref_axis',(0.47354689410563,0.254189745109288,0.843291712614435));
#17435=DIRECTION('center_axis',(-0.4309815049242,-0.768119965562789,0.473546894105633));
#17436=DIRECTION('ref_axis',(0.47354689410563,0.254189745109288,0.843291712614435));
#17437=DIRECTION('',(-0.4309815049242,-0.768119965562789,0.473546894105633));
#17438=DIRECTION('center_axis',(0.4309815049242,0.768119965562789,-0.473546894105633));
#17439=DIRECTION('ref_axis',(-0.76811996556279,0.587689792309766,0.254189745109285));
#17440=DIRECTION('center_axis',(0.4309815049242,0.768119965562789,-0.473546894105633));
#17441=DIRECTION('ref_axis',(-0.76811996556279,0.587689792309766,0.254189745109285));
#17442=DIRECTION('center_axis',(-0.76811996556279,0.587689792309766,0.254189745109285));
#17443=DIRECTION('ref_axis',(0.4309815049242,0.768119965562789,-0.473546894105633));
#17444=DIRECTION('',(0.4309815049242,0.768119965562789,-0.473546894105633));
#17445=DIRECTION('',(0.473546894105632,0.254189745109287,0.843291712614434));
#17446=DIRECTION('',(0.4309815049242,0.768119965562789,-0.473546894105633));
#17447=DIRECTION('center_axis',(0.473546894105632,0.254189745109286,0.843291712614434));
#17448=DIRECTION('ref_axis',(0.4309815049242,0.768119965562789,-0.473546894105633));
#17449=DIRECTION('',(0.76811996556279,-0.587689792309766,-0.254189745109284));
#17450=DIRECTION('',(-0.4309815049242,-0.768119965562789,0.473546894105633));
#17451=DIRECTION('',(0.4309815049242,0.768119965562789,-0.473546894105633));
#17452=DIRECTION('center_axis',(-0.76811996556279,0.587689792309766,0.254189745109285));
#17453=DIRECTION('ref_axis',(0.4309815049242,0.768119965562789,-0.473546894105633));
#17454=DIRECTION('',(0.4309815049242,0.768119965562789,-0.473546894105633));
#17455=DIRECTION('',(0.473546894105632,0.254189745109287,0.843291712614434));
#17456=DIRECTION('center_axis',(-0.473546894105632,-0.254189745109286,-0.843291712614434));
#17457=DIRECTION('ref_axis',(0.76811996556279,-0.587689792309766,-0.254189745109285));
#17458=DIRECTION('',(0.4309815049242,0.768119965562789,-0.473546894105633));
#17459=DIRECTION('',(-0.76811996556279,0.587689792309766,0.254189745109284));
#17460=DIRECTION('center_axis',(-0.364685089938824,0.628286844373993,0.687212067969474));
#17461=DIRECTION('ref_axis',(0.4309815049242,0.768119965562789,-0.473546894105633));
#17462=DIRECTION('',(0.4309815049242,0.768119965562789,-0.473546894105633));
#17463=DIRECTION('',(0.825384593743779,-0.123480199588392,0.550901908437453));
#17464=DIRECTION('center_axis',(0.0449396061089009,-0.542406212931599,-0.838913542610905));
#17465=DIRECTION('ref_axis',(0.901241018937803,-0.340275210200539,0.268286054626271));
#17466=DIRECTION('',(-0.4309815049242,-0.768119965562789,0.473546894105633));
#17467=DIRECTION('',(-0.901241018937803,0.340275210200539,-0.268286054626271));
#17468=DIRECTION('center_axis',(-0.76811996556279,0.587689792309766,0.254189745109285));
#17469=DIRECTION('ref_axis',(0.4309815049242,0.768119965562789,-0.473546894105633));
#17470=DIRECTION('',(0.473546894105632,0.254189745109287,0.843291712614434));
#17471=DIRECTION('',(0.4309815049242,0.768119965562789,-0.473546894105633));
#17472=DIRECTION('center_axis',(-0.473546894105632,-0.254189745109286,-0.843291712614434));
#17473=DIRECTION('ref_axis',(0.76811996556279,-0.587689792309766,-0.254189745109285));
#17474=DIRECTION('',(0.4309815049242,0.768119965562789,-0.473546894105633));
#17475=DIRECTION('',(-0.76811996556279,0.587689792309766,0.254189745109284));
#17476=DIRECTION('center_axis',(0.76811996556279,-0.587689792309766,-0.254189745109285));
#17477=DIRECTION('ref_axis',(-0.473546894105632,-0.254189745109287,-0.843291712614434));
#17478=DIRECTION('',(0.4309815049242,0.768119965562789,-0.473546894105633));
#17479=DIRECTION('',(-0.473546894105632,-0.254189745109287,-0.843291712614434));
#17480=DIRECTION('center_axis',(-0.825384593743779,0.123480199588392,-0.550901908437453));
#17481=DIRECTION('ref_axis',(-0.4309815049242,-0.768119965562789,0.473546894105633));
#17482=DIRECTION('',(0.4309815049242,0.768119965562789,-0.473546894105633));
#17483=DIRECTION('',(-0.364685089938824,0.628286844373994,0.687212067969474));
#17484=DIRECTION('center_axis',(0.901241018937803,-0.340275210200539,0.268286054626271));
#17485=DIRECTION('ref_axis',(-0.4309815049242,-0.768119965562789,0.473546894105633));
#17486=DIRECTION('',(-0.4309815049242,-0.768119965562789,0.473546894105633));
#17487=DIRECTION('',(0.0449396061089009,-0.542406212931599,-0.838913542610905));
#17488=DIRECTION('center_axis',(-0.473546894105632,-0.254189745109286,-0.843291712614434));
#17489=DIRECTION('ref_axis',(0.76811996556279,-0.587689792309766,-0.254189745109285));
#17490=DIRECTION('',(-0.76811996556279,0.587689792309766,0.254189745109284));
#17491=DIRECTION('',(0.4309815049242,0.768119965562789,-0.473546894105633));
#17492=DIRECTION('center_axis',(0.76811996556279,-0.587689792309766,-0.254189745109285));
#17493=DIRECTION('ref_axis',(-0.473546894105632,-0.254189745109287,-0.843291712614434));
#17494=DIRECTION('',(0.4309815049242,0.768119965562789,-0.473546894105633));
#17495=DIRECTION('',(-0.473546894105632,-0.254189745109287,-0.843291712614434));
#17496=DIRECTION('center_axis',(0.473546894105632,0.254189745109286,0.843291712614434));
#17497=DIRECTION('ref_axis',(0.4309815049242,0.768119965562789,-0.473546894105633));
#17498=DIRECTION('',(0.4309815049242,0.768119965562789,-0.473546894105633));
#17499=DIRECTION('',(0.76811996556279,-0.587689792309766,-0.254189745109284));
#17500=DIRECTION('center_axis',(0.364685089938824,-0.628286844373994,-0.687212067969474));
#17501=DIRECTION('ref_axis',(-0.825384593743779,0.123480199588392,-0.550901908437453));
#17502=DIRECTION('',(0.4309815049242,0.768119965562789,-0.473546894105633));
#17503=DIRECTION('',(-0.825384593743779,0.123480199588392,-0.550901908437453));
#17504=DIRECTION('center_axis',(-0.0449396061089009,0.542406212931599,0.838913542610905));
#17505=DIRECTION('ref_axis',(0.4309815049242,0.768119965562789,-0.473546894105633));
#17506=DIRECTION('',(-0.4309815049242,-0.768119965562789,0.473546894105633));
#17507=DIRECTION('',(0.901241018937803,-0.340275210200539,0.268286054626271));
#17508=DIRECTION('center_axis',(0.76811996556279,-0.587689792309766,-0.254189745109285));
#17509=DIRECTION('ref_axis',(-0.473546894105632,-0.254189745109287,-0.843291712614434));
#17510=DIRECTION('',(-0.473546894105632,-0.254189745109287,-0.843291712614434));
#17511=DIRECTION('',(0.4309815049242,0.768119965562789,-0.473546894105633));
#17512=DIRECTION('center_axis',(0.473546894105632,0.254189745109286,0.843291712614434));
#17513=DIRECTION('ref_axis',(0.4309815049242,0.768119965562789,-0.473546894105633));
#17514=DIRECTION('',(0.76811996556279,-0.587689792309766,-0.254189745109284));
#17515=DIRECTION('center_axis',(0.4309815049242,0.768119965562789,-0.473546894105633));
#17516=DIRECTION('ref_axis',(0.76811996556279,-0.587689792309766,-0.254189745109285));
#17517=DIRECTION('',(-0.0449396061089009,0.542406212931599,0.838913542610905));
#17518=DIRECTION('',(0.364685089938824,-0.628286844373994,-0.687212067969474));
#17519=DIRECTION('center_axis',(0.825384593743779,-0.123480199588392,0.550901908437453));
#17520=DIRECTION('ref_axis',(-0.4309815049242,-0.768119965562789,0.473546894105633));
#17521=DIRECTION('',(0.4309815049242,0.768119965562789,-0.473546894105633));
#17522=DIRECTION('center_axis',(-0.901241018937803,0.340275210200539,-0.268286054626271));
#17523=DIRECTION('ref_axis',(-0.4309815049242,-0.768119965562789,0.473546894105633));
#33916=CARTESIAN_POINT('',(0.,0.,0.));
#33917=CARTESIAN_POINT('Origin',(-28.393108630048,72.7321117214098,30.9925849618393));
#33918=CARTESIAN_POINT('',(-38.9069263049545,56.3529534297169,37.0903559934943));
#33919=CARTESIAN_POINT('Origin',(-37.012738728532,57.369712410154,40.463522843952));
#33920=CARTESIAN_POINT('',(-39.7810443854308,54.7950500343233,38.0508053338062));
#33921=CARTESIAN_POINT('',(-30.2872962064705,71.7153527409726,27.6194181113816));
#33922=CARTESIAN_POINT('Origin',(-37.8868568090083,55.8118090147604,41.423972184264));
#33923=CARTESIAN_POINT('Origin',(-34.9009293544028,61.1335002414122,38.1431430628339));
#33924=CARTESIAN_POINT('',(-40.232869135087,56.4700997583121,41.8610879399662));
#33925=CARTESIAN_POINT('',(-39.6882902068655,56.7624179651878,42.8308734094728));
#33926=CARTESIAN_POINT('Origin',(-36.6676052751974,62.4851867637248,38.7277794765853));
#33927=CARTESIAN_POINT('',(-38.7873697728656,55.7663207511003,42.6252145919964));
#33928=CARTESIAN_POINT('Origin',(-34.6286398902921,61.2796593448501,38.6280357975872));
#33929=CARTESIAN_POINT('',(-38.7033067843916,56.8717526272238,43.7448778970514));
#33930=CARTESIAN_POINT('Origin',(-35.3279590748654,61.2947308388206,38.016022662737));
#33931=CARTESIAN_POINT('',(-38.296523342403,55.6344840136914,42.8580939635258));
#33932=CARTESIAN_POINT('Origin',(-34.5098422368239,61.0749923461824,38.4041736673213));
#33933=CARTESIAN_POINT('',(-37.5464148739375,56.1871303837669,43.8470743034192));
#33934=CARTESIAN_POINT('Origin',(-35.3425983346016,61.4714218719905,38.2893021662718));
#33935=CARTESIAN_POINT('',(-36.6630769135403,55.5112871226107,43.5547560965436));
#33936=CARTESIAN_POINT('Origin',(-33.8117714979599,61.7181366551636,40.0827140018471));
#33937=CARTESIAN_POINT('',(-37.4131853820058,54.9586407525351,42.5657757566501));
#33938=CARTESIAN_POINT('Origin',(-34.4592603742044,60.7955786108343,37.9969839593961));
#33939=CARTESIAN_POINT('',(-35.8766253111206,54.7090541915238,42.8094596350493));
#33940=CARTESIAN_POINT('Origin',(-34.92222282311,61.3905053805684,38.5406405225208));
#33941=CARTESIAN_POINT('',(-37.2967369646954,54.6258352478992,42.1319276178937));
#33942=CARTESIAN_POINT('Origin',(-34.7281327675399,60.8358027888048,37.8175254188111));
#33943=CARTESIAN_POINT('',(-36.1549383652767,54.0590449205628,41.6616005819702));
#33944=CARTESIAN_POINT('Origin',(-34.6286398902921,61.2796593448501,38.6280357975872));
#33945=CARTESIAN_POINT('',(-36.6995172934982,53.7667267136871,40.6918151124636));
#33946=CARTESIAN_POINT('Origin',(-33.1342534336086,59.7818137190999,37.5585066490826));
#33947=CARTESIAN_POINT('',(-37.8413158929169,54.3335170410235,41.1621421483871));
#33948=CARTESIAN_POINT('Origin',(-35.1732188185136,60.9873411379744,37.6582503280806));
#33949=CARTESIAN_POINT('',(-37.6192778814294,53.7736359295216,39.7061461326282));
#33950=CARTESIAN_POINT('Origin',(-34.4738996339406,60.972269644004,38.2702634629306));
#33951=CARTESIAN_POINT('',(-38.3321623233795,54.4653537784324,40.9292627768577));
#33952=CARTESIAN_POINT('Origin',(-35.292016471982,61.1920081366421,37.8821124583463));
#33953=CARTESIAN_POINT('',(-38.8413926264262,54.342014295108,39.6756142185172));
#33954=CARTESIAN_POINT('Origin',(-34.4592603742044,60.7955786108343,37.9969839593961));
#33955=CARTESIAN_POINT('',(-39.7247305868234,55.0178575562642,39.9679324253928));
#33956=CARTESIAN_POINT('Origin',(-35.9900872108458,60.5488638276609,36.2035721238207));
#33957=CARTESIAN_POINT('',(-39.2155002837767,55.1411970395887,41.2215809837334));
#33958=CARTESIAN_POINT('Origin',(-35.3425983346016,61.4714218719905,38.2893021662718));
#33959=CARTESIAN_POINT('',(-40.4459593547004,55.9363343652216,40.6415643946303));
#33960=CARTESIAN_POINT('Origin',(-34.8796358856957,60.8764951022562,37.7456456031473));
#33961=CARTESIAN_POINT('',(-39.3319487010871,55.4740025442247,41.6554291224898));
#33962=CARTESIAN_POINT('Origin',(-35.0737259412659,61.4311976940199,38.468760706857));
#33963=CARTESIAN_POINT('Origin',(-35.1732188185136,60.9873411379744,37.6582503280806));
#33964=CARTESIAN_POINT('Origin',(-36.8403461265623,57.6769603963792,40.2741040863097));
#33965=CARTESIAN_POINT('',(-38.0545418955644,56.8104949709136,38.6082810762002));
#33966=CARTESIAN_POINT('Origin',(-37.012738728532,57.369712410154,40.463522843952));
#33967=CARTESIAN_POINT('',(-37.696662681666,57.2124706447442,38.7603610476862));
#33968=CARTESIAN_POINT('Origin',(-37.8821492935947,57.1177429571387,38.418862318558));
#33969=CARTESIAN_POINT('Origin',(-36.8442301901646,57.6700379953797,40.2783717549553));
#33970=CARTESIAN_POINT('Origin',(-36.8442301901646,57.6700379953797,40.2783717549553));
#33971=CARTESIAN_POINT('',(-37.4056077410637,57.7224461315386,38.4608120751962));
#33972=CARTESIAN_POINT('',(-37.696662681666,57.2124706447442,38.7603610476862));
#33973=CARTESIAN_POINT('',(-35.7148085556595,58.6300306164513,41.471785135086));
#33974=CARTESIAN_POINT('Origin',(-36.5602081483616,58.1762383739949,39.9662986051411));
#33975=CARTESIAN_POINT('Origin',(-36.5602081483616,58.1762383739949,39.9662986051411));
#33976=CARTESIAN_POINT('Origin',(-36.5602081483616,58.1762383739949,39.9662986051411));
#33977=CARTESIAN_POINT('',(-37.0547713564024,58.4743848476173,37.7824909411013));
#33978=CARTESIAN_POINT('',(-35.1605837799799,59.4911438280544,41.155657791559));
#33979=CARTESIAN_POINT('Origin',(-36.1076775681912,58.9827643378359,39.4690743663302));
#33980=CARTESIAN_POINT('',(-35.7148085556595,58.6300306164513,41.471785135086));
#33981=CARTESIAN_POINT('Origin',(-36.1076775681912,58.9827643378359,39.4690743663302));
#33982=CARTESIAN_POINT('Origin',(-28.393108630048,72.7321117214098,30.9925849618393));
#33983=CARTESIAN_POINT('',(-29.3402024182593,72.2237322311912,29.3060015366105));
#33984=CARTESIAN_POINT('Origin',(-28.393108630048,72.7321117214098,30.9925849618393));
#33985=CARTESIAN_POINT('',(-29.3402024182593,72.2237322311912,29.3060015366105));
#33986=CARTESIAN_POINT('Origin',(-29.9293485611736,73.9074913060293,31.5009644520579));
#33987=CARTESIAN_POINT('Origin',(-40.0852185907832,59.7204715793931,41.4802818243891));
#33988=CARTESIAN_POINT('Origin',(-39.1543717028682,54.3387298731897,43.2616154689789));
#33989=CARTESIAN_POINT('',(-37.6311300310271,56.8203861500479,42.1269838523944));
#33990=CARTESIAN_POINT('',(-38.9671726962921,54.4392142568033,43.5949792241218));
#33991=CARTESIAN_POINT('',(-37.001460645271,57.1583790767479,43.2482983015114));
#33992=CARTESIAN_POINT('',(-37.8183290376032,56.7199017664344,41.7936200972515));
#33993=CARTESIAN_POINT('',(-38.337503310536,54.7772071835033,44.7162936732388));
#33994=CARTESIAN_POINT('Origin',(-40.4793786434641,55.3524947649241,43.7000927792924));
#33995=CARTESIAN_POINT('',(-39.143335978199,57.7336666581687,42.232097407565));
#33996=CARTESIAN_POINT('',(-38.1219764614898,56.9522228874568,41.894104480865));
#33997=CARTESIAN_POINT('',(-39.143335978199,57.7336666581687,42.232097407565));
#33998=CARTESIAN_POINT('',(-39.4580191267548,54.5710509942122,43.3620998525924));
#33999=CARTESIAN_POINT('',(-40.4793786434641,55.3524947649241,43.7000927792924));
#34000=CARTESIAN_POINT('Origin',(-41.0239575716855,55.0601765580484,42.7303073097858));
#34001=CARTESIAN_POINT('',(-39.6879149064205,57.4413484512931,41.2623119380584));
#34002=CARTESIAN_POINT('',(-41.0239575716855,55.0601765580484,42.7303073097858));
#34003=CARTESIAN_POINT('',(-39.6879149064205,57.4413484512931,41.2623119380584));
#34004=CARTESIAN_POINT('Origin',(-39.6989506310897,54.0464116663141,42.2918299994723));
#34005=CARTESIAN_POINT('',(-38.6665553897112,56.6599046805812,40.9243190113584));
#34006=CARTESIAN_POINT('',(-40.0025980549763,54.2787327873365,42.3923143830858));
#34007=CARTESIAN_POINT('',(-38.3629079658247,56.4275835595587,40.8238346277449));
#34008=CARTESIAN_POINT('Origin',(-41.2696592085703,54.4682892260227,41.5466160105783));
#34009=CARTESIAN_POINT('',(-39.9336165433053,56.8494611192673,40.0786206388509));
#34010=CARTESIAN_POINT('',(-41.2696592085703,54.4682892260227,41.5466160105783));
#34011=CARTESIAN_POINT('',(-39.9336165433053,56.8494611192673,40.0786206388509));
#34012=CARTESIAN_POINT('Origin',(-39.2572816508911,53.708490035736,42.1456708960345));
#34013=CARTESIAN_POINT('',(-38.5501069724008,56.3270991759452,40.490470872602));
#34014=CARTESIAN_POINT('',(-39.8861496376659,53.9459272827006,41.9584662443294));
#34015=CARTESIAN_POINT('',(-37.9212389856261,56.0896619289806,40.677675524307));
#34016=CARTESIAN_POINT('Origin',(-40.5158190234219,53.6079343560005,40.8371517952124));
#34017=CARTESIAN_POINT('',(-39.1797763581569,55.9891062492452,39.369156423485));
#34018=CARTESIAN_POINT('',(-39.1797763581569,55.9891062492452,39.369156423485));
#34019=CARTESIAN_POINT('',(-40.5158190234219,53.6079343560005,40.8371517952124));
#34020=CARTESIAN_POINT('Origin',(-39.6324810630247,52.9320910948443,40.5448335883368));
#34021=CARTESIAN_POINT('',(-38.2964383977597,55.313262988089,39.0768382166093));
#34022=CARTESIAN_POINT('',(-39.6324810630247,52.9320910948443,40.5448335883368));
#34023=CARTESIAN_POINT('',(-38.2964383977597,55.313262988089,39.0768382166093));
#34024=CARTESIAN_POINT('Origin',(-38.8156126706925,53.3705684051578,41.9995117925966));
#34025=CARTESIAN_POINT('',(-37.6667690120036,55.651255914789,40.1981526657263));
#34026=CARTESIAN_POINT('',(-39.0028116772686,53.2700840215443,41.6661480374538));
#34027=CARTESIAN_POINT('',(-37.4795700054275,55.7517402984025,40.5315164208692));
#34028=CARTESIAN_POINT('Origin',(-38.4429777352992,52.3055907903227,40.6111977485762));
#34029=CARTESIAN_POINT('',(-37.1069350700342,54.6867626835674,39.1432023768487));
#34030=CARTESIAN_POINT('',(-38.4429777352992,52.3055907903227,40.6111977485762));
#34031=CARTESIAN_POINT('',(-37.1069350700342,54.6867626835674,39.1432023768487));
#34032=CARTESIAN_POINT('Origin',(-38.5433232065818,53.5167275085957,42.48440452735));
#34033=CARTESIAN_POINT('',(-37.1759225815409,55.51941917738,40.4310320372557));
#34034=CARTESIAN_POINT('',(-38.511965246806,53.1382472841354,41.8990274089831));
#34035=CARTESIAN_POINT('',(-37.2072805413167,55.8978994018403,41.0164091556225));
#34036=CARTESIAN_POINT('Origin',(-37.4906057300967,52.3568035134235,41.5610344822831));
#34037=CARTESIAN_POINT('',(-36.1545630648317,54.7379754066681,40.0930391105557));
#34038=CARTESIAN_POINT('',(-36.1545630648317,54.7379754066681,40.0930391105557));
#34039=CARTESIAN_POINT('',(-37.4906057300967,52.3568035134235,41.5610344822831));
#34040=CARTESIAN_POINT('Origin',(-36.9460268018752,52.6491217202992,42.5308199517897));
#34041=CARTESIAN_POINT('',(-35.6099841366102,55.0302936135438,41.0628245800623));
#34042=CARTESIAN_POINT('',(-36.9460268018752,52.6491217202992,42.5308199517897));
#34043=CARTESIAN_POINT('',(-35.6099841366102,55.0302936135438,41.0628245800623));
#34044=CARTESIAN_POINT('Origin',(-38.271033742471,53.6628866120335,42.9692972621033));
#34045=CARTESIAN_POINT('',(-36.6313436533195,55.8117373842557,41.4008175067623));
#34046=CARTESIAN_POINT('',(-37.9673863185845,53.4305654910111,42.8688128784897));
#34047=CARTESIAN_POINT('',(-36.934991077206,56.0440585052782,41.5013018903758));
#34048=CARTESIAN_POINT('Origin',(-36.7003251649905,53.2410090523249,43.7145112509973));
#34049=CARTESIAN_POINT('',(-35.3642824997255,55.6221809455696,42.2465158792698));
#34050=CARTESIAN_POINT('',(-36.7003251649905,53.2410090523249,43.7145112509973));
#34051=CARTESIAN_POINT('',(-35.3642824997255,55.6221809455696,42.2465158792698));
#34052=CARTESIAN_POINT('Origin',(-38.7127027226696,54.0008082426116,43.1154563655411));
#34053=CARTESIAN_POINT('',(-36.7477920706299,56.1445428888917,41.8346656455187));
#34054=CARTESIAN_POINT('',(-38.0838347358949,53.763370995647,43.3026610172461));
#34055=CARTESIAN_POINT('',(-37.3766600574046,56.3819801358563,41.6474609938136));
#34056=CARTESIAN_POINT('Origin',(-37.4541653501388,54.101363922347,44.4239754663631));
#34057=CARTESIAN_POINT('',(-36.1181226848738,56.4825358155917,42.9559800946357));
#34058=CARTESIAN_POINT('',(-36.1181226848738,56.4825358155917,42.9559800946357));
#34059=CARTESIAN_POINT('',(-37.4541653501388,54.101363922347,44.4239754663631));
#34060=CARTESIAN_POINT('Origin',(-38.337503310536,54.7772071835033,44.7162936732388));
#34061=CARTESIAN_POINT('',(-37.001460645271,57.1583790767479,43.2482983015114));
#34062=CARTESIAN_POINT('Origin',(-36.1181226848738,56.4825358155917,42.9559800946357));
#34063=CARTESIAN_POINT('',(-38.1909639729965,57.7848793812695,43.181934141272));
#34064=CARTESIAN_POINT('',(-38.090618501714,56.5737426629966,41.3087273624982));
#34065=CARTESIAN_POINT('',(-38.1909639729965,57.7848793812695,43.181934141272));
#34066=CARTESIAN_POINT('Origin',(-39.5270066382616,55.4037074880248,44.6499295129994));
#34067=CARTESIAN_POINT('',(-39.5270066382616,55.4037074880248,44.6499295129994));
#34068=CARTESIAN_POINT('Origin',(-39.426661166979,54.1925707697519,42.7767227342256));
#62949=UNCERTAINTY_MEASURE_WITH_UNIT(LENGTH_MEASURE(0.01),#62975,
'DISTANCE_ACCURACY_VALUE',
'Maximum model space distance between geometric entities at asserted c
onnectivities');
#62960=UNCERTAINTY_MEASURE_WITH_UNIT(LENGTH_MEASURE(0.01),#62975,
'DISTANCE_ACCURACY_VALUE',
'Maximum model space distance between geometric entities at asserted c
onnectivities');
#62963=(
GEOMETRIC_REPRESENTATION_CONTEXT(3)
GLOBAL_UNCERTAINTY_ASSIGNED_CONTEXT((#62949))
GLOBAL_UNIT_ASSIGNED_CONTEXT((#62975,#62977,#62978))
REPRESENTATION_CONTEXT('','3D')
);
#62974=(
GEOMETRIC_REPRESENTATION_CONTEXT(3)
GLOBAL_UNCERTAINTY_ASSIGNED_CONTEXT((#62960))
GLOBAL_UNIT_ASSIGNED_CONTEXT((#62975,#62977,#62978))
REPRESENTATION_CONTEXT('','3D')
);
#62975=(
LENGTH_UNIT()
NAMED_UNIT(*)
SI_UNIT(.MILLI.,.METRE.)
);
#62977=(
NAMED_UNIT(*)
PLANE_ANGLE_UNIT()
SI_UNIT($,.RADIAN.)
);
#62978=(
NAMED_UNIT(*)
SI_UNIT($,.STERADIAN.)
SOLID_ANGLE_UNIT()
);
#62981=SHAPE_DEFINITION_REPRESENTATION(#62994,#63022);
#62994=PRODUCT_DEFINITION_SHAPE('',$,#63036);
#63022=SHAPE_REPRESENTATION('',(#15471),#62963);
#63033=PRODUCT_DEFINITION_CONTEXT('part definition',#63074,'design');
#63036=PRODUCT_DEFINITION('DIN 7985 M4x20','DIN 7985 M4x20',#63049,#63033);
#63049=PRODUCT_DEFINITION_FORMATION('',$,#63078);
#63074=APPLICATION_CONTEXT(
'Core Data for Automotive Mechanical Design Process');
#63075=PRODUCT_CONTEXT('part definition',#63074,'mechanical');
#63078=PRODUCT('DIN 7985 M4x20','DIN 7985 M4x20',$,(#63075));
#63090=PRESENTATION_STYLE_ASSIGNMENT((#63092));
#63092=SURFACE_STYLE_USAGE(.BOTH.,#63094);
#63094=SURFACE_SIDE_STYLE('',(#63096));
#63096=SURFACE_STYLE_FILL_AREA(#63098);
#63098=FILL_AREA_STYLE('Opaque(202,209,238)',(#63100));
#63100=FILL_AREA_STYLE_COLOUR('Opaque(202,209,238)',#63102);
#63102=COLOUR_RGB('Opaque(202,209,238)', 0.66274510, 0.83137255, 0.94901961);
ENDSEC;
END-ISO-10303-21;
